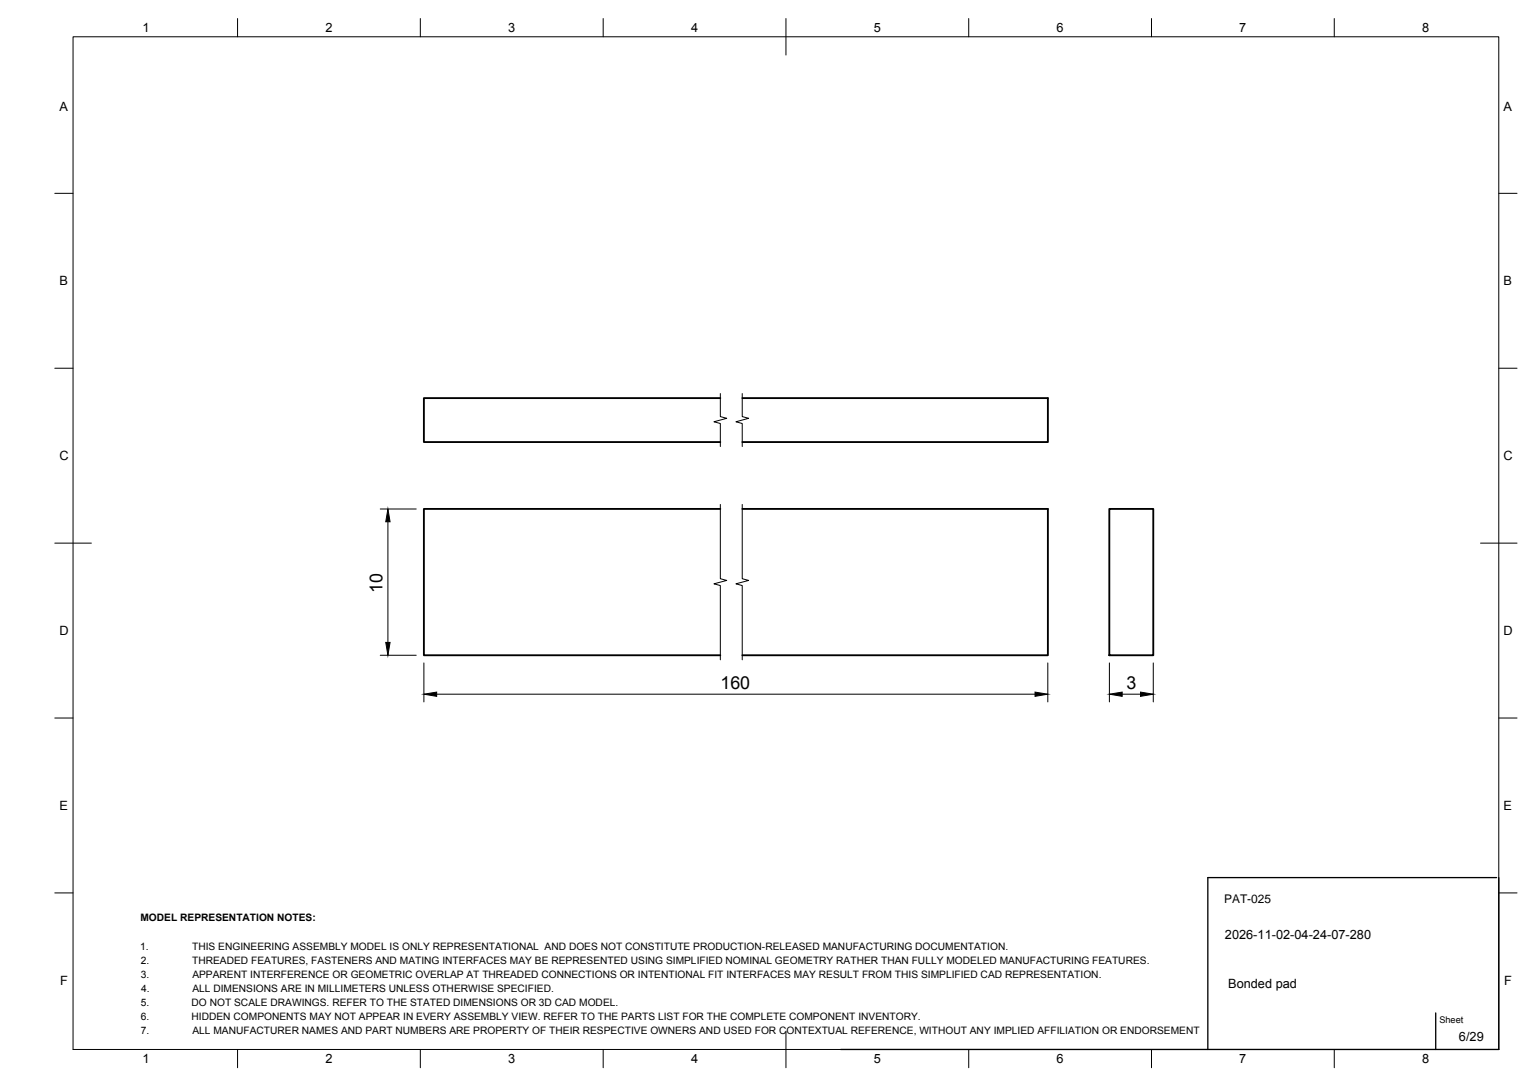
ISO-10303-21;
HEADER;
/* Generated by software containing ST-Developer
 * from STEP Tools, Inc. (www.steptools.com) 
 */

FILE_DESCRIPTION(
/* description */ ('Counter shaft with two pulleys and keyed hub'),
/* implementation_level */ '2;1');

FILE_NAME(
/* name */ 'Bonded pad.step',
/* time_stamp */ '2026-10-27T10:46:10-07:00',
/* author */ (''),
/* organization */ (''),
/* preprocessor_version */ 'ST-DEVELOPER v20.2',
/* originating_system */ 'Autodesk Translation Framework v15.17.0.0',
/* authorisation */ '');

FILE_SCHEMA (('AUTOMOTIVE_DESIGN { 1 0 10303 214 3 1 1 }'));
ENDSEC;

DATA;
#10=MECHANICAL_DESIGN_GEOMETRIC_PRESENTATION_REPRESENTATION('',(#291),#10821);
#241=SHAPE_REPRESENTATION_RELATIONSHIP('SRR','None',#10927,#266);
#266=ADVANCED_BREP_SHAPE_REPRESENTATION('',(#317),#10795);
#291=STYLED_ITEM('',(#11149),#317);
#317=MANIFOLD_SOLID_BREP('Body1',#5574);
#437=PLANE('',#5899);
#438=PLANE('',#5900);
#439=PLANE('',#5901);
#440=PLANE('',#5902);
#441=PLANE('',#5903);
#442=PLANE('',#5904);
#598=FACE_OUTER_BOUND('',#920,.T.);
#599=FACE_OUTER_BOUND('',#921,.T.);
#600=FACE_OUTER_BOUND('',#922,.T.);
#601=FACE_OUTER_BOUND('',#923,.T.);
#602=FACE_OUTER_BOUND('',#924,.T.);
#603=FACE_OUTER_BOUND('',#925,.T.);
#920=EDGE_LOOP('',(#3677,#3678,#3679,#3680));
#921=EDGE_LOOP('',(#3681,#3682,#3683,#3684));
#922=EDGE_LOOP('',(#3685,#3686,#3687,#3688));
#923=EDGE_LOOP('',(#3689,#3690,#3691,#3692));
#924=EDGE_LOOP('',(#3693,#3694,#3695,#3696));
#925=EDGE_LOOP('',(#3697,#3698,#3699,#3700));
#1323=LINE('',#8369,#1712);
#1324=LINE('',#8371,#1713);
#1325=LINE('',#8373,#1714);
#1326=LINE('',#8374,#1715);
#1327=LINE('',#8377,#1716);
#1328=LINE('',#8379,#1717);
#1329=LINE('',#8380,#1718);
#1330=LINE('',#8383,#1719);
#1331=LINE('',#8385,#1720);
#1332=LINE('',#8386,#1721);
#1333=LINE('',#8388,#1722);
#1334=LINE('',#8389,#1723);
#1712=VECTOR('',#6621,1.);
#1713=VECTOR('',#6622,1.);
#1714=VECTOR('',#6623,1.);
#1715=VECTOR('',#6624,1.);
#1716=VECTOR('',#6627,1.);
#1717=VECTOR('',#6628,1.);
#1718=VECTOR('',#6629,1.);
#1719=VECTOR('',#6632,1.);
#1720=VECTOR('',#6633,1.);
#1721=VECTOR('',#6634,1.);
#1722=VECTOR('',#6637,1.);
#1723=VECTOR('',#6638,1.);
#2400=VERTEX_POINT('',#8367);
#2401=VERTEX_POINT('',#8368);
#2402=VERTEX_POINT('',#8370);
#2403=VERTEX_POINT('',#8372);
#2404=VERTEX_POINT('',#8376);
#2405=VERTEX_POINT('',#8378);
#2406=VERTEX_POINT('',#8382);
#2407=VERTEX_POINT('',#8384);
#2911=EDGE_CURVE('',#2400,#2401,#1323,.T.);
#2912=EDGE_CURVE('',#2401,#2402,#1324,.T.);
#2913=EDGE_CURVE('',#2403,#2402,#1325,.T.);
#2914=EDGE_CURVE('',#2400,#2403,#1326,.T.);
#2915=EDGE_CURVE('',#2404,#2400,#1327,.T.);
#2916=EDGE_CURVE('',#2405,#2403,#1328,.T.);
#2917=EDGE_CURVE('',#2404,#2405,#1329,.T.);
#2918=EDGE_CURVE('',#2406,#2404,#1330,.T.);
#2919=EDGE_CURVE('',#2407,#2405,#1331,.T.);
#2920=EDGE_CURVE('',#2406,#2407,#1332,.T.);
#2921=EDGE_CURVE('',#2401,#2406,#1333,.T.);
#2922=EDGE_CURVE('',#2402,#2407,#1334,.T.);
#3677=ORIENTED_EDGE('',*,*,#2911,.T.);
#3678=ORIENTED_EDGE('',*,*,#2912,.T.);
#3679=ORIENTED_EDGE('',*,*,#2913,.F.);
#3680=ORIENTED_EDGE('',*,*,#2914,.F.);
#3681=ORIENTED_EDGE('',*,*,#2915,.T.);
#3682=ORIENTED_EDGE('',*,*,#2914,.T.);
#3683=ORIENTED_EDGE('',*,*,#2916,.F.);
#3684=ORIENTED_EDGE('',*,*,#2917,.F.);
#3685=ORIENTED_EDGE('',*,*,#2918,.T.);
#3686=ORIENTED_EDGE('',*,*,#2917,.T.);
#3687=ORIENTED_EDGE('',*,*,#2919,.F.);
#3688=ORIENTED_EDGE('',*,*,#2920,.F.);
#3689=ORIENTED_EDGE('',*,*,#2921,.T.);
#3690=ORIENTED_EDGE('',*,*,#2920,.T.);
#3691=ORIENTED_EDGE('',*,*,#2922,.F.);
#3692=ORIENTED_EDGE('',*,*,#2912,.F.);
#3693=ORIENTED_EDGE('',*,*,#2922,.T.);
#3694=ORIENTED_EDGE('',*,*,#2919,.T.);
#3695=ORIENTED_EDGE('',*,*,#2916,.T.);
#3696=ORIENTED_EDGE('',*,*,#2913,.T.);
#3697=ORIENTED_EDGE('',*,*,#2921,.F.);
#3698=ORIENTED_EDGE('',*,*,#2911,.F.);
#3699=ORIENTED_EDGE('',*,*,#2915,.F.);
#3700=ORIENTED_EDGE('',*,*,#2918,.F.);
#5269=ADVANCED_FACE('',(#598),#437,.T.);
#5270=ADVANCED_FACE('',(#599),#438,.T.);
#5271=ADVANCED_FACE('',(#600),#439,.T.);
#5272=ADVANCED_FACE('',(#601),#440,.T.);
#5273=ADVANCED_FACE('',(#602),#441,.T.);
#5274=ADVANCED_FACE('',(#603),#442,.F.);
#5574=CLOSED_SHELL('',(#5269,#5270,#5271,#5272,#5273,#5274));
#5898=AXIS2_PLACEMENT_3D('',#8365,#6617,#6618);
#5899=AXIS2_PLACEMENT_3D('',#8366,#6619,#6620);
#5900=AXIS2_PLACEMENT_3D('',#8375,#6625,#6626);
#5901=AXIS2_PLACEMENT_3D('',#8381,#6630,#6631);
#5902=AXIS2_PLACEMENT_3D('',#8387,#6635,#6636);
#5903=AXIS2_PLACEMENT_3D('',#8390,#6639,#6640);
#5904=AXIS2_PLACEMENT_3D('',#8391,#6641,#6642);
#6617=DIRECTION('axis',(0.,0.,1.));
#6618=DIRECTION('refdir',(1.,0.,0.));
#6619=DIRECTION('center_axis',(0.,1.,0.));
#6620=DIRECTION('ref_axis',(-1.,0.,0.));
#6621=DIRECTION('',(-1.,0.,0.));
#6622=DIRECTION('',(0.,0.,1.));
#6623=DIRECTION('',(-1.,0.,0.));
#6624=DIRECTION('',(0.,0.,1.));
#6625=DIRECTION('center_axis',(1.,0.,0.));
#6626=DIRECTION('ref_axis',(0.,1.,0.));
#6627=DIRECTION('',(0.,1.,0.));
#6628=DIRECTION('',(0.,1.,0.));
#6629=DIRECTION('',(0.,0.,1.));
#6630=DIRECTION('center_axis',(0.,-1.,0.));
#6631=DIRECTION('ref_axis',(1.,0.,0.));
#6632=DIRECTION('',(1.,0.,0.));
#6633=DIRECTION('',(1.,0.,0.));
#6634=DIRECTION('',(0.,0.,1.));
#6635=DIRECTION('center_axis',(-1.,0.,0.));
#6636=DIRECTION('ref_axis',(0.,-1.,0.));
#6637=DIRECTION('',(0.,-1.,0.));
#6638=DIRECTION('',(0.,-1.,0.));
#6639=DIRECTION('center_axis',(0.,0.,1.));
#6640=DIRECTION('ref_axis',(1.,0.,0.));
#6641=DIRECTION('center_axis',(0.,0.,1.));
#6642=DIRECTION('ref_axis',(1.,0.,0.));
#8365=CARTESIAN_POINT('',(0.,0.,0.));
#8366=CARTESIAN_POINT('Origin',(8.,-6.,-0.3));
#8367=CARTESIAN_POINT('',(8.,-6.,-0.3));
#8368=CARTESIAN_POINT('',(-8.,-6.,-0.3));
#8369=CARTESIAN_POINT('',(8.,-6.,-0.3));
#8370=CARTESIAN_POINT('',(-8.,-6.,0.));
#8371=CARTESIAN_POINT('',(-8.,-6.,-0.3));
#8372=CARTESIAN_POINT('',(8.,-6.,0.));
#8373=CARTESIAN_POINT('',(8.,-6.,0.));
#8374=CARTESIAN_POINT('',(8.,-6.,-0.3));
#8375=CARTESIAN_POINT('Origin',(8.,-7.,-0.3));
#8376=CARTESIAN_POINT('',(8.,-7.,-0.3));
#8377=CARTESIAN_POINT('',(8.,-7.,-0.3));
#8378=CARTESIAN_POINT('',(8.,-7.,0.));
#8379=CARTESIAN_POINT('',(8.,-7.,0.));
#8380=CARTESIAN_POINT('',(8.,-7.,-0.3));
#8381=CARTESIAN_POINT('Origin',(-8.,-7.,-0.3));
#8382=CARTESIAN_POINT('',(-8.,-7.,-0.3));
#8383=CARTESIAN_POINT('',(-8.,-7.,-0.3));
#8384=CARTESIAN_POINT('',(-8.,-7.,0.));
#8385=CARTESIAN_POINT('',(-8.,-7.,0.));
#8386=CARTESIAN_POINT('',(-8.,-7.,-0.3));
#8387=CARTESIAN_POINT('Origin',(-8.,-6.,-0.3));
#8388=CARTESIAN_POINT('',(-8.,-6.,-0.3));
#8389=CARTESIAN_POINT('',(-8.,-6.,0.));
#8390=CARTESIAN_POINT('Origin',(0.,-6.5,0.));
#8391=CARTESIAN_POINT('Origin',(0.,-6.5,-0.3));
#10765=UNCERTAINTY_MEASURE_WITH_UNIT(LENGTH_MEASURE(0.001),#10822,
'DISTANCE_ACCURACY_VALUE',
'Maximum model space distance between geometric entities at asserted c
onnectivities');
#10791=UNCERTAINTY_MEASURE_WITH_UNIT(LENGTH_MEASURE(0.001),#10822,
'DISTANCE_ACCURACY_VALUE',
'Maximum model space distance between geometric entities at asserted c
onnectivities');
#10795=(
GEOMETRIC_REPRESENTATION_CONTEXT(3)
GLOBAL_UNCERTAINTY_ASSIGNED_CONTEXT((#10765))
GLOBAL_UNIT_ASSIGNED_CONTEXT((#10822,#10824,#10825))
REPRESENTATION_CONTEXT('','3D')
);
#10821=(
GEOMETRIC_REPRESENTATION_CONTEXT(3)
GLOBAL_UNCERTAINTY_ASSIGNED_CONTEXT((#10791))
GLOBAL_UNIT_ASSIGNED_CONTEXT((#10822,#10824,#10825))
REPRESENTATION_CONTEXT('','3D')
);
#10822=(
LENGTH_UNIT()
NAMED_UNIT(*)
SI_UNIT(.CENTI.,.METRE.)
);
#10824=(
NAMED_UNIT(*)
PLANE_ANGLE_UNIT()
SI_UNIT($,.RADIAN.)
);
#10825=(
NAMED_UNIT(*)
SI_UNIT($,.STERADIAN.)
SOLID_ANGLE_UNIT()
);
#10829=SHAPE_DEFINITION_REPRESENTATION(#10858,#10927);
#10858=PRODUCT_DEFINITION_SHAPE('',$,#10957);
#10927=SHAPE_REPRESENTATION('',(#5898),#10795);
#10953=PRODUCT_DEFINITION_CONTEXT('part definition',#11042,'design');
#10957=PRODUCT_DEFINITION('Bonded pad','Bonded pad',#10986,#10953);
#10986=PRODUCT_DEFINITION_FORMATION('',$,#11047);
#11042=APPLICATION_CONTEXT(
'Core Data for Automotive Mechanical Design Process');
#11043=PRODUCT_CONTEXT('part definition',#11042,'mechanical');
#11047=PRODUCT('Bonded pad','Bonded pad','Bonded pad',(#11043));
#11143=COLOUR_RGB('Off White',0.89,0.88,0.83);
#11144=FILL_AREA_STYLE_COLOUR('',#11143);
#11145=FILL_AREA_STYLE('',(#11144));
#11146=SURFACE_STYLE_FILL_AREA(#11145);
#11147=SURFACE_SIDE_STYLE('',(#11146));
#11148=SURFACE_STYLE_USAGE(.BOTH.,#11147);
#11149=PRESENTATION_STYLE_ASSIGNMENT((#11148));
ENDSEC;
END-ISO-10303-21;
